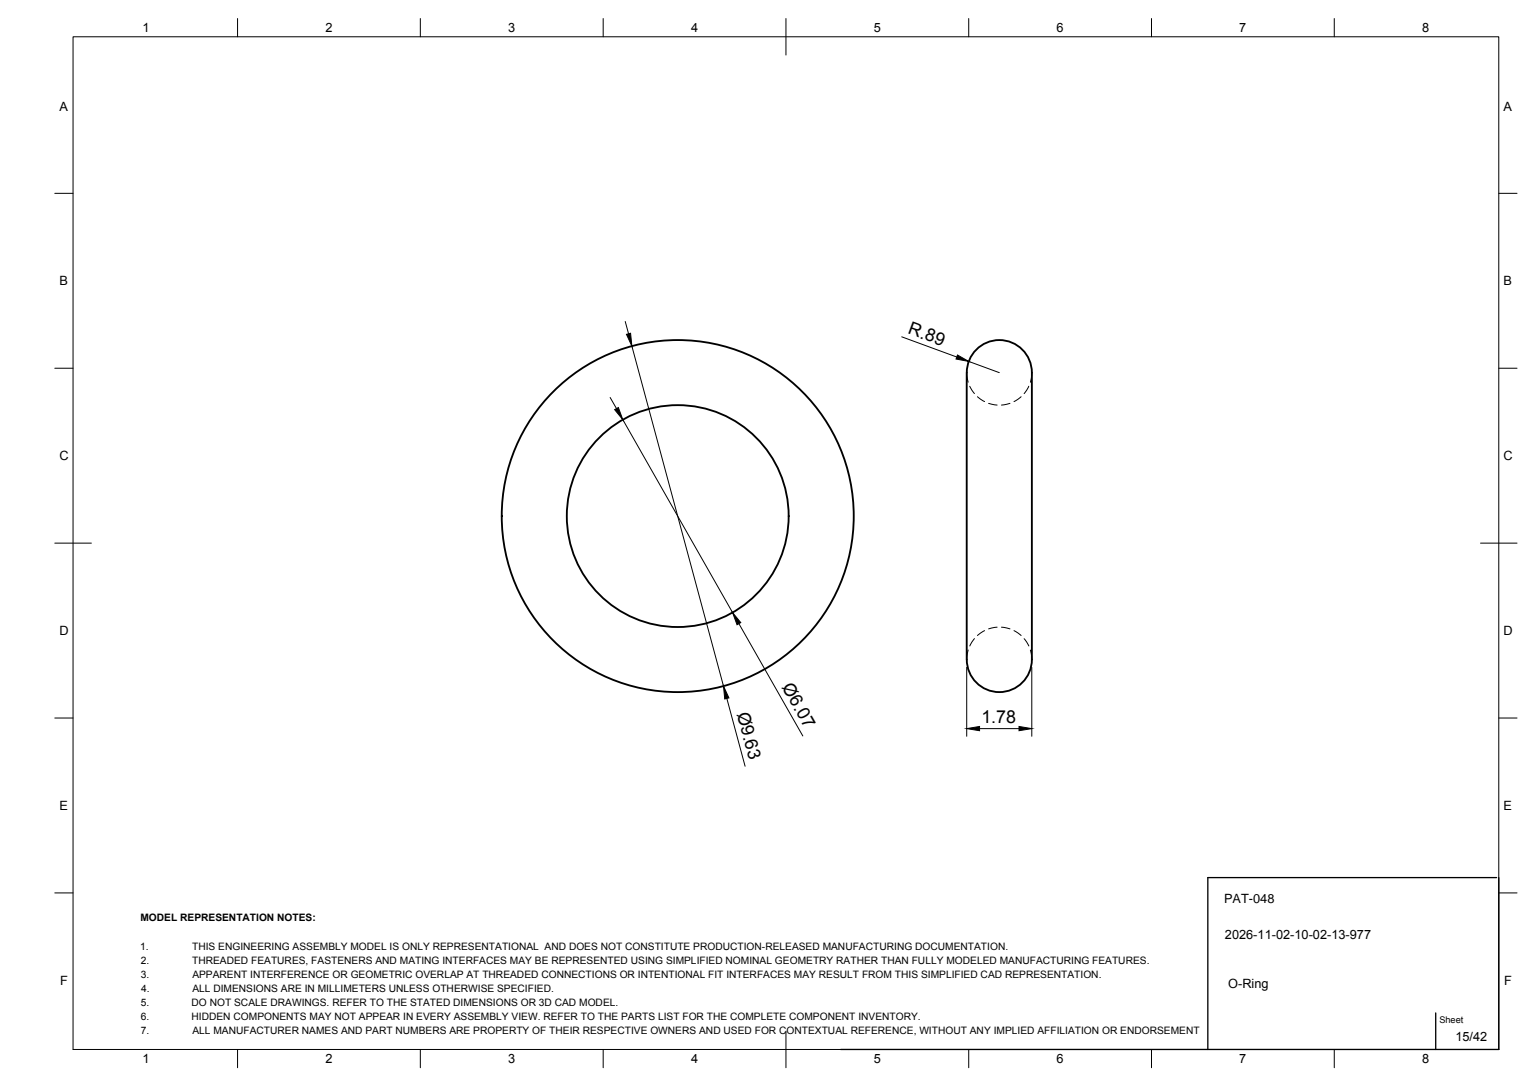
ISO-10303-21;
HEADER;
/* Generated by software containing ST-Developer
 * from STEP Tools, Inc. (www.steptools.com) 
 */

FILE_DESCRIPTION(
/* description */ ('Guided pneumatic stop gate'),
/* implementation_level */ '2;1');

FILE_NAME(
/* name */ 'O-Ring.step',
/* time_stamp */ '2026-10-27T21:43:45-07:00',
/* author */ (''),
/* organization */ (''),
/* preprocessor_version */ 'ST-DEVELOPER v20.2',
/* originating_system */ 'Autodesk Translation Framework v15.17.0.0',
/* authorisation */ '');

FILE_SCHEMA (('AUTOMOTIVE_DESIGN { 1 0 10303 214 3 1 1 }'));
ENDSEC;

DATA;
#10=MECHANICAL_DESIGN_GEOMETRIC_PRESENTATION_REPRESENTATION('',(#548),#14392);
#43=TOROIDAL_SURFACE('',#8768,0.3925,0.089);
#464=SHAPE_REPRESENTATION_RELATIONSHIP('SRR','None',#14599,#506);
#506=ADVANCED_BREP_SHAPE_REPRESENTATION('',(#589),#14361);
#548=STYLED_ITEM('',(#14898),#589);
#589=MANIFOLD_SOLID_BREP('Body1',#7889);
#1321=FACE_OUTER_BOUND('',#1872,.T.);
#1872=EDGE_LOOP('',(#6118,#6119,#6120,#6121));
#3516=CIRCLE('',#8769,0.089);
#3517=CIRCLE('',#8770,0.3035);
#3991=VERTEX_POINT('',#12798);
#4757=EDGE_CURVE('',#3991,#3991,#3516,.T.);
#4758=EDGE_CURVE('',#3991,#3991,#3517,.T.);
#6118=ORIENTED_EDGE('',*,*,#4757,.F.);
#6119=ORIENTED_EDGE('',*,*,#4758,.T.);
#6120=ORIENTED_EDGE('',*,*,#4757,.T.);
#6121=ORIENTED_EDGE('',*,*,#4758,.F.);
#7603=ADVANCED_FACE('',(#1321),#43,.T.);
#7889=CLOSED_SHELL('',(#7603));
#8767=AXIS2_PLACEMENT_3D('',#12796,#10386,#10387);
#8768=AXIS2_PLACEMENT_3D('',#12797,#10388,#10389);
#8769=AXIS2_PLACEMENT_3D('',#12799,#10390,#10391);
#8770=AXIS2_PLACEMENT_3D('',#12800,#10392,#10393);
#10386=DIRECTION('axis',(0.,0.,1.));
#10387=DIRECTION('refdir',(1.,0.,0.));
#10388=DIRECTION('center_axis',(0.,-1.,0.));
#10389=DIRECTION('ref_axis',(0.,0.,-1.));
#10390=DIRECTION('center_axis',(-1.,0.,-1.22464679914735E-16));
#10391=DIRECTION('ref_axis',(-1.22464679914735E-16,0.,1.));
#10392=DIRECTION('center_axis',(0.,1.,0.));
#10393=DIRECTION('ref_axis',(0.,0.,-1.));
#12796=CARTESIAN_POINT('',(0.,0.,0.));
#12797=CARTESIAN_POINT('Origin',(0.,0.,0.));
#12798=CARTESIAN_POINT('',(-3.71680303541222E-17,-1.08993565124114E-17,
0.3035));
#12799=CARTESIAN_POINT('Origin',(-4.80673868665336E-17,0.,0.3925));
#12800=CARTESIAN_POINT('Origin',(0.,1.08993565124114E-17,0.));
#14313=UNCERTAINTY_MEASURE_WITH_UNIT(LENGTH_MEASURE(0.001),#14393,
'DISTANCE_ACCURACY_VALUE',
'Maximum model space distance between geometric entities at asserted c
onnectivities');
#14344=UNCERTAINTY_MEASURE_WITH_UNIT(LENGTH_MEASURE(0.001),#14393,
'DISTANCE_ACCURACY_VALUE',
'Maximum model space distance between geometric entities at asserted c
onnectivities');
#14361=(
GEOMETRIC_REPRESENTATION_CONTEXT(3)
GLOBAL_UNCERTAINTY_ASSIGNED_CONTEXT((#14313))
GLOBAL_UNIT_ASSIGNED_CONTEXT((#14393,#14395,#14396))
REPRESENTATION_CONTEXT('','3D')
);
#14392=(
GEOMETRIC_REPRESENTATION_CONTEXT(3)
GLOBAL_UNCERTAINTY_ASSIGNED_CONTEXT((#14344))
GLOBAL_UNIT_ASSIGNED_CONTEXT((#14393,#14395,#14396))
REPRESENTATION_CONTEXT('','3D')
);
#14393=(
LENGTH_UNIT()
NAMED_UNIT(*)
SI_UNIT(.CENTI.,.METRE.)
);
#14395=(
NAMED_UNIT(*)
PLANE_ANGLE_UNIT()
SI_UNIT($,.RADIAN.)
);
#14396=(
NAMED_UNIT(*)
SI_UNIT($,.STERADIAN.)
SOLID_ANGLE_UNIT()
);
#14413=SHAPE_DEFINITION_REPRESENTATION(#14462,#14599);
#14462=PRODUCT_DEFINITION_SHAPE('',$,#14647);
#14599=SHAPE_REPRESENTATION('',(#8767),#14361);
#14630=PRODUCT_DEFINITION_CONTEXT('part definition',#14773,'design');
#14647=PRODUCT_DEFINITION('O-Ring','O-Ring',#14694,#14630);
#14694=PRODUCT_DEFINITION_FORMATION('',$,#14791);
#14773=APPLICATION_CONTEXT(
'Core Data for Automotive Mechanical Design Process');
#14774=PRODUCT_CONTEXT('part definition',#14773,'mechanical');
#14791=PRODUCT('O-Ring','O-Ring','O-Ring',(#14774));
#14892=COLOUR_RGB('Black',0.12,0.14,0.17);
#14893=FILL_AREA_STYLE_COLOUR('',#14892);
#14894=FILL_AREA_STYLE('',(#14893));
#14895=SURFACE_STYLE_FILL_AREA(#14894);
#14896=SURFACE_SIDE_STYLE('',(#14895));
#14897=SURFACE_STYLE_USAGE(.BOTH.,#14896);
#14898=PRESENTATION_STYLE_ASSIGNMENT((#14897));
ENDSEC;
END-ISO-10303-21;
